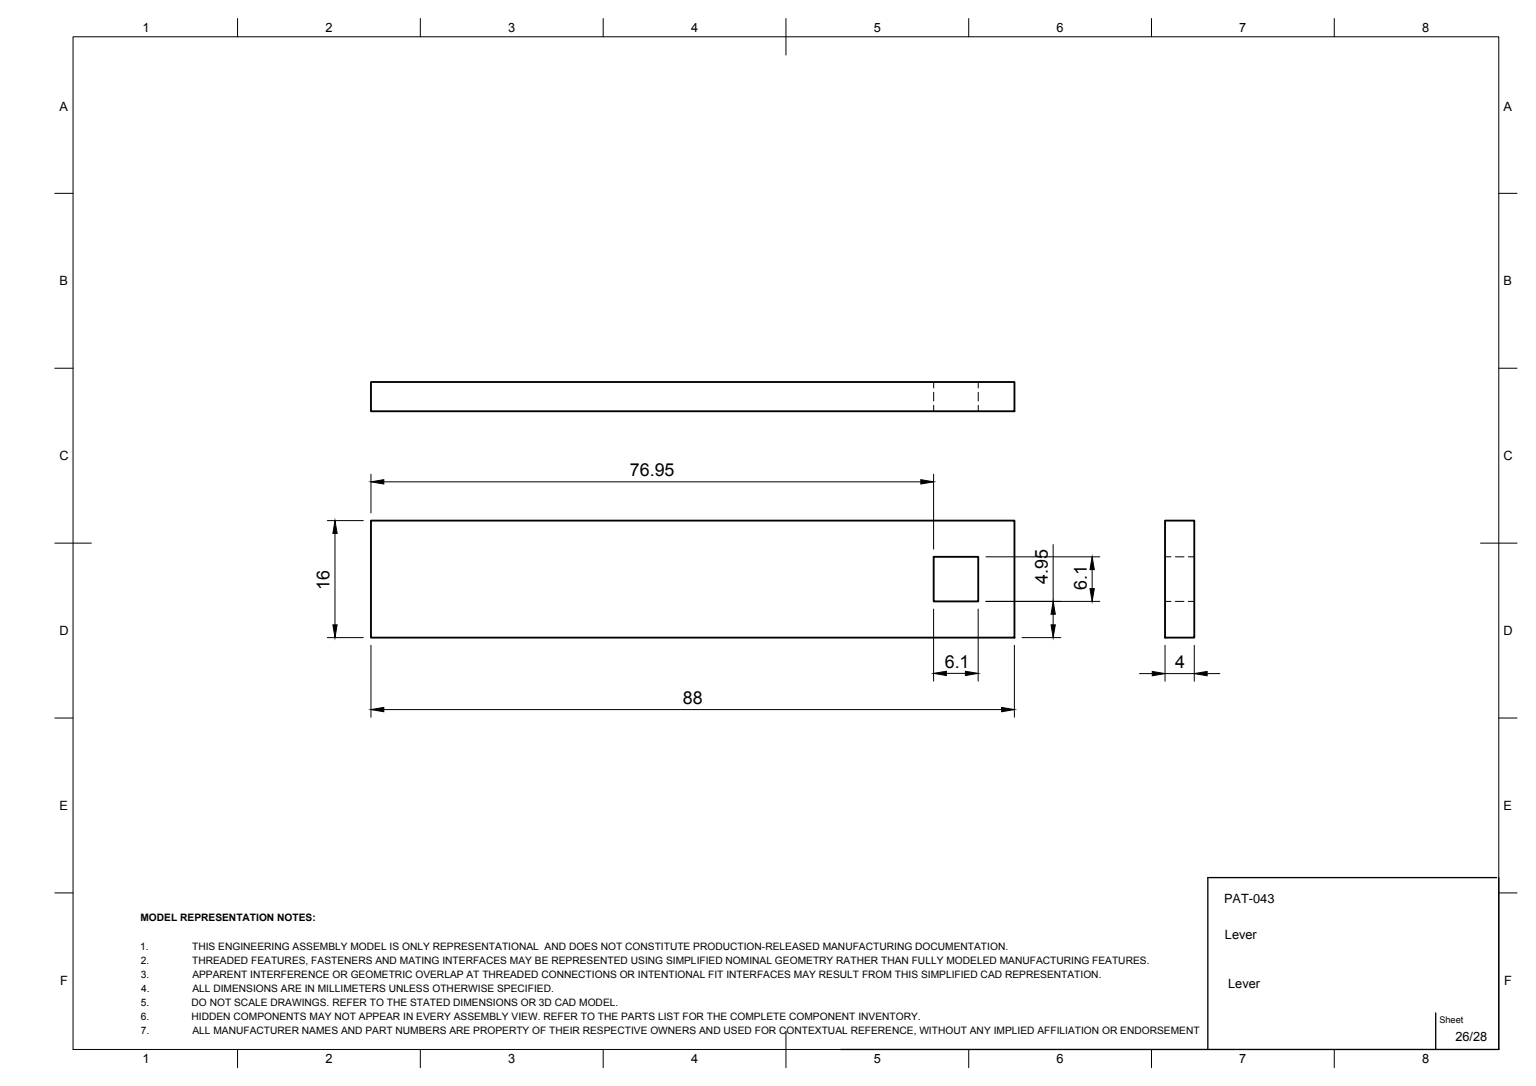
ISO-10303-21;
HEADER;
/* Generated by software containing ST-Developer
 * from STEP Tools, Inc. (www.steptools.com) 
 */

FILE_DESCRIPTION(
/* description */ ('Four-valve pipe header'),
/* implementation_level */ '2;1');

FILE_NAME(
/* name */ 'Lever.step',
/* time_stamp */ '2026-10-29T16:56:19-07:00',
/* author */ (''),
/* organization */ (''),
/* preprocessor_version */ 'ST-DEVELOPER v20.2',
/* originating_system */ 'Autodesk Translation Framework v15.17.0.0',
/* authorisation */ '');

FILE_SCHEMA (('AUTOMOTIVE_DESIGN { 1 0 10303 214 3 1 1 }'));
ENDSEC;

DATA;
#10=MECHANICAL_DESIGN_GEOMETRIC_PRESENTATION_REPRESENTATION('',(#355),#10119);
#303=SHAPE_REPRESENTATION_RELATIONSHIP('SRR','None',#10266,#329);
#329=ADVANCED_BREP_SHAPE_REPRESENTATION('',(#379),#10115);
#355=STYLED_ITEM('',(#10484),#379);
#379=MANIFOLD_SOLID_BREP('Body1',#5603);
#530=FACE_BOUND('',#1488,.T.);
#531=FACE_BOUND('',#1490,.T.);
#718=PLANE('',#6463);
#719=PLANE('',#6464);
#720=PLANE('',#6465);
#721=PLANE('',#6466);
#722=PLANE('',#6467);
#723=PLANE('',#6468);
#724=PLANE('',#6469);
#725=PLANE('',#6470);
#726=PLANE('',#6471);
#727=PLANE('',#6472);
#1043=FACE_OUTER_BOUND('',#1479,.T.);
#1044=FACE_OUTER_BOUND('',#1480,.T.);
#1045=FACE_OUTER_BOUND('',#1481,.T.);
#1046=FACE_OUTER_BOUND('',#1482,.T.);
#1047=FACE_OUTER_BOUND('',#1483,.T.);
#1048=FACE_OUTER_BOUND('',#1484,.T.);
#1049=FACE_OUTER_BOUND('',#1485,.T.);
#1050=FACE_OUTER_BOUND('',#1486,.T.);
#1051=FACE_OUTER_BOUND('',#1487,.T.);
#1052=FACE_OUTER_BOUND('',#1489,.T.);
#1479=EDGE_LOOP('',(#5005,#5006,#5007,#5008));
#1480=EDGE_LOOP('',(#5009,#5010,#5011,#5012));
#1481=EDGE_LOOP('',(#5013,#5014,#5015,#5016));
#1482=EDGE_LOOP('',(#5017,#5018,#5019,#5020));
#1483=EDGE_LOOP('',(#5021,#5022,#5023,#5024));
#1484=EDGE_LOOP('',(#5025,#5026,#5027,#5028));
#1485=EDGE_LOOP('',(#5029,#5030,#5031,#5032));
#1486=EDGE_LOOP('',(#5033,#5034,#5035,#5036));
#1487=EDGE_LOOP('',(#5037,#5038,#5039,#5040));
#1488=EDGE_LOOP('',(#5041,#5042,#5043,#5044));
#1489=EDGE_LOOP('',(#5045,#5046,#5047,#5048));
#1490=EDGE_LOOP('',(#5049,#5050,#5051,#5052));
#1877=LINE('',#9847,#2295);
#1878=LINE('',#9849,#2296);
#1879=LINE('',#9851,#2297);
#1880=LINE('',#9852,#2298);
#1881=LINE('',#9855,#2299);
#1882=LINE('',#9857,#2300);
#1883=LINE('',#9858,#2301);
#1884=LINE('',#9861,#2302);
#1885=LINE('',#9863,#2303);
#1886=LINE('',#9864,#2304);
#1887=LINE('',#9866,#2305);
#1888=LINE('',#9867,#2306);
#1889=LINE('',#9871,#2307);
#1890=LINE('',#9873,#2308);
#1891=LINE('',#9875,#2309);
#1892=LINE('',#9876,#2310);
#1893=LINE('',#9879,#2311);
#1894=LINE('',#9881,#2312);
#1895=LINE('',#9882,#2313);
#1896=LINE('',#9885,#2314);
#1897=LINE('',#9887,#2315);
#1898=LINE('',#9888,#2316);
#1899=LINE('',#9890,#2317);
#1900=LINE('',#9891,#2318);
#2295=VECTOR('',#8064,1.);
#2296=VECTOR('',#8065,1.);
#2297=VECTOR('',#8066,1.);
#2298=VECTOR('',#8067,1.);
#2299=VECTOR('',#8070,1.);
#2300=VECTOR('',#8071,1.);
#2301=VECTOR('',#8072,1.);
#2302=VECTOR('',#8075,1.);
#2303=VECTOR('',#8076,1.);
#2304=VECTOR('',#8077,1.);
#2305=VECTOR('',#8080,1.);
#2306=VECTOR('',#8081,1.);
#2307=VECTOR('',#8084,1.);
#2308=VECTOR('',#8085,1.);
#2309=VECTOR('',#8086,1.);
#2310=VECTOR('',#8087,1.);
#2311=VECTOR('',#8090,1.);
#2312=VECTOR('',#8091,1.);
#2313=VECTOR('',#8092,1.);
#2314=VECTOR('',#8095,1.);
#2315=VECTOR('',#8096,1.);
#2316=VECTOR('',#8097,1.);
#2317=VECTOR('',#8100,1.);
#2318=VECTOR('',#8101,1.);
#2990=VERTEX_POINT('',#9845);
#2991=VERTEX_POINT('',#9846);
#2992=VERTEX_POINT('',#9848);
#2993=VERTEX_POINT('',#9850);
#2994=VERTEX_POINT('',#9854);
#2995=VERTEX_POINT('',#9856);
#2996=VERTEX_POINT('',#9860);
#2997=VERTEX_POINT('',#9862);
#2998=VERTEX_POINT('',#9869);
#2999=VERTEX_POINT('',#9870);
#3000=VERTEX_POINT('',#9872);
#3001=VERTEX_POINT('',#9874);
#3002=VERTEX_POINT('',#9878);
#3003=VERTEX_POINT('',#9880);
#3004=VERTEX_POINT('',#9884);
#3005=VERTEX_POINT('',#9886);
#3669=EDGE_CURVE('',#2990,#2991,#1877,.T.);
#3670=EDGE_CURVE('',#2992,#2990,#1878,.T.);
#3671=EDGE_CURVE('',#2993,#2992,#1879,.T.);
#3672=EDGE_CURVE('',#2993,#2991,#1880,.T.);
#3673=EDGE_CURVE('',#2991,#2994,#1881,.T.);
#3674=EDGE_CURVE('',#2995,#2993,#1882,.T.);
#3675=EDGE_CURVE('',#2995,#2994,#1883,.T.);
#3676=EDGE_CURVE('',#2994,#2996,#1884,.T.);
#3677=EDGE_CURVE('',#2997,#2995,#1885,.T.);
#3678=EDGE_CURVE('',#2997,#2996,#1886,.T.);
#3679=EDGE_CURVE('',#2996,#2990,#1887,.T.);
#3680=EDGE_CURVE('',#2992,#2997,#1888,.T.);
#3681=EDGE_CURVE('',#2998,#2999,#1889,.T.);
#3682=EDGE_CURVE('',#2999,#3000,#1890,.T.);
#3683=EDGE_CURVE('',#3001,#3000,#1891,.T.);
#3684=EDGE_CURVE('',#2998,#3001,#1892,.T.);
#3685=EDGE_CURVE('',#3002,#2998,#1893,.T.);
#3686=EDGE_CURVE('',#3003,#3001,#1894,.T.);
#3687=EDGE_CURVE('',#3002,#3003,#1895,.T.);
#3688=EDGE_CURVE('',#3004,#3002,#1896,.T.);
#3689=EDGE_CURVE('',#3005,#3003,#1897,.T.);
#3690=EDGE_CURVE('',#3004,#3005,#1898,.T.);
#3691=EDGE_CURVE('',#2999,#3004,#1899,.T.);
#3692=EDGE_CURVE('',#3000,#3005,#1900,.T.);
#5005=ORIENTED_EDGE('',*,*,#3669,.F.);
#5006=ORIENTED_EDGE('',*,*,#3670,.F.);
#5007=ORIENTED_EDGE('',*,*,#3671,.F.);
#5008=ORIENTED_EDGE('',*,*,#3672,.T.);
#5009=ORIENTED_EDGE('',*,*,#3673,.F.);
#5010=ORIENTED_EDGE('',*,*,#3672,.F.);
#5011=ORIENTED_EDGE('',*,*,#3674,.F.);
#5012=ORIENTED_EDGE('',*,*,#3675,.T.);
#5013=ORIENTED_EDGE('',*,*,#3676,.F.);
#5014=ORIENTED_EDGE('',*,*,#3675,.F.);
#5015=ORIENTED_EDGE('',*,*,#3677,.F.);
#5016=ORIENTED_EDGE('',*,*,#3678,.T.);
#5017=ORIENTED_EDGE('',*,*,#3679,.F.);
#5018=ORIENTED_EDGE('',*,*,#3678,.F.);
#5019=ORIENTED_EDGE('',*,*,#3680,.F.);
#5020=ORIENTED_EDGE('',*,*,#3670,.T.);
#5021=ORIENTED_EDGE('',*,*,#3681,.T.);
#5022=ORIENTED_EDGE('',*,*,#3682,.T.);
#5023=ORIENTED_EDGE('',*,*,#3683,.F.);
#5024=ORIENTED_EDGE('',*,*,#3684,.F.);
#5025=ORIENTED_EDGE('',*,*,#3685,.T.);
#5026=ORIENTED_EDGE('',*,*,#3684,.T.);
#5027=ORIENTED_EDGE('',*,*,#3686,.F.);
#5028=ORIENTED_EDGE('',*,*,#3687,.F.);
#5029=ORIENTED_EDGE('',*,*,#3688,.T.);
#5030=ORIENTED_EDGE('',*,*,#3687,.T.);
#5031=ORIENTED_EDGE('',*,*,#3689,.F.);
#5032=ORIENTED_EDGE('',*,*,#3690,.F.);
#5033=ORIENTED_EDGE('',*,*,#3691,.T.);
#5034=ORIENTED_EDGE('',*,*,#3690,.T.);
#5035=ORIENTED_EDGE('',*,*,#3692,.F.);
#5036=ORIENTED_EDGE('',*,*,#3682,.F.);
#5037=ORIENTED_EDGE('',*,*,#3692,.T.);
#5038=ORIENTED_EDGE('',*,*,#3689,.T.);
#5039=ORIENTED_EDGE('',*,*,#3686,.T.);
#5040=ORIENTED_EDGE('',*,*,#3683,.T.);
#5041=ORIENTED_EDGE('',*,*,#3676,.T.);
#5042=ORIENTED_EDGE('',*,*,#3679,.T.);
#5043=ORIENTED_EDGE('',*,*,#3669,.T.);
#5044=ORIENTED_EDGE('',*,*,#3673,.T.);
#5045=ORIENTED_EDGE('',*,*,#3691,.F.);
#5046=ORIENTED_EDGE('',*,*,#3681,.F.);
#5047=ORIENTED_EDGE('',*,*,#3685,.F.);
#5048=ORIENTED_EDGE('',*,*,#3688,.F.);
#5049=ORIENTED_EDGE('',*,*,#3677,.T.);
#5050=ORIENTED_EDGE('',*,*,#3674,.T.);
#5051=ORIENTED_EDGE('',*,*,#3671,.T.);
#5052=ORIENTED_EDGE('',*,*,#3680,.T.);
#5543=ADVANCED_FACE('',(#1043),#718,.F.);
#5544=ADVANCED_FACE('',(#1044),#719,.F.);
#5545=ADVANCED_FACE('',(#1045),#720,.F.);
#5546=ADVANCED_FACE('',(#1046),#721,.F.);
#5547=ADVANCED_FACE('',(#1047),#722,.T.);
#5548=ADVANCED_FACE('',(#1048),#723,.T.);
#5549=ADVANCED_FACE('',(#1049),#724,.T.);
#5550=ADVANCED_FACE('',(#1050),#725,.T.);
#5551=ADVANCED_FACE('',(#1051,#530),#726,.T.);
#5552=ADVANCED_FACE('',(#1052,#531),#727,.F.);
#5603=CLOSED_SHELL('',(#5543,#5544,#5545,#5546,#5547,#5548,#5549,#5550,
#5551,#5552));
#6462=AXIS2_PLACEMENT_3D('',#9843,#8060,#8061);
#6463=AXIS2_PLACEMENT_3D('',#9844,#8062,#8063);
#6464=AXIS2_PLACEMENT_3D('',#9853,#8068,#8069);
#6465=AXIS2_PLACEMENT_3D('',#9859,#8073,#8074);
#6466=AXIS2_PLACEMENT_3D('',#9865,#8078,#8079);
#6467=AXIS2_PLACEMENT_3D('',#9868,#8082,#8083);
#6468=AXIS2_PLACEMENT_3D('',#9877,#8088,#8089);
#6469=AXIS2_PLACEMENT_3D('',#9883,#8093,#8094);
#6470=AXIS2_PLACEMENT_3D('',#9889,#8098,#8099);
#6471=AXIS2_PLACEMENT_3D('',#9892,#8102,#8103);
#6472=AXIS2_PLACEMENT_3D('',#9893,#8104,#8105);
#8060=DIRECTION('axis',(0.,0.,1.));
#8061=DIRECTION('refdir',(1.,0.,0.));
#8062=DIRECTION('center_axis',(0.,-1.,0.));
#8063=DIRECTION('ref_axis',(1.,0.,0.));
#8064=DIRECTION('',(-1.,0.,0.));
#8065=DIRECTION('',(0.,0.,1.));
#8066=DIRECTION('',(1.,0.,0.));
#8067=DIRECTION('',(0.,0.,1.));
#8068=DIRECTION('center_axis',(-1.,0.,0.));
#8069=DIRECTION('ref_axis',(0.,-1.,0.));
#8070=DIRECTION('',(0.,1.,0.));
#8071=DIRECTION('',(0.,-1.,0.));
#8072=DIRECTION('',(0.,0.,1.));
#8073=DIRECTION('center_axis',(0.,1.,0.));
#8074=DIRECTION('ref_axis',(-1.,0.,0.));
#8075=DIRECTION('',(1.,0.,0.));
#8076=DIRECTION('',(-1.,0.,0.));
#8077=DIRECTION('',(0.,0.,1.));
#8078=DIRECTION('center_axis',(1.,0.,0.));
#8079=DIRECTION('ref_axis',(0.,1.,0.));
#8080=DIRECTION('',(0.,-1.,0.));
#8081=DIRECTION('',(0.,1.,0.));
#8082=DIRECTION('center_axis',(0.,1.,0.));
#8083=DIRECTION('ref_axis',(-1.,0.,0.));
#8084=DIRECTION('',(-1.,0.,0.));
#8085=DIRECTION('',(0.,0.,1.));
#8086=DIRECTION('',(-1.,0.,0.));
#8087=DIRECTION('',(0.,0.,1.));
#8088=DIRECTION('center_axis',(1.,0.,0.));
#8089=DIRECTION('ref_axis',(0.,1.,0.));
#8090=DIRECTION('',(0.,1.,0.));
#8091=DIRECTION('',(0.,1.,0.));
#8092=DIRECTION('',(0.,0.,1.));
#8093=DIRECTION('center_axis',(0.,-1.,0.));
#8094=DIRECTION('ref_axis',(1.,0.,0.));
#8095=DIRECTION('',(1.,0.,0.));
#8096=DIRECTION('',(1.,0.,0.));
#8097=DIRECTION('',(0.,0.,1.));
#8098=DIRECTION('center_axis',(-1.,0.,0.));
#8099=DIRECTION('ref_axis',(0.,-1.,0.));
#8100=DIRECTION('',(0.,-1.,0.));
#8101=DIRECTION('',(0.,-1.,0.));
#8102=DIRECTION('center_axis',(0.,0.,1.));
#8103=DIRECTION('ref_axis',(1.,0.,0.));
#8104=DIRECTION('center_axis',(0.,0.,1.));
#8105=DIRECTION('ref_axis',(1.,0.,0.));
#9843=CARTESIAN_POINT('',(0.,0.,0.));
#9844=CARTESIAN_POINT('Origin',(-0.305,-0.305,8.9));
#9845=CARTESIAN_POINT('',(0.305,-0.305,9.4));
#9846=CARTESIAN_POINT('',(-0.305,-0.305,9.4));
#9847=CARTESIAN_POINT('',(1.6475,-0.305,9.4));
#9848=CARTESIAN_POINT('',(0.305,-0.305,9.));
#9849=CARTESIAN_POINT('',(0.305,-0.305,8.9));
#9850=CARTESIAN_POINT('',(-0.305,-0.305,9.));
#9851=CARTESIAN_POINT('',(1.6475,-0.305,9.));
#9852=CARTESIAN_POINT('',(-0.305,-0.305,8.9));
#9853=CARTESIAN_POINT('Origin',(-0.305,0.305,8.9));
#9854=CARTESIAN_POINT('',(-0.305,0.305,9.4));
#9855=CARTESIAN_POINT('',(-0.305,0.1525,9.4));
#9856=CARTESIAN_POINT('',(-0.305,0.305,9.));
#9857=CARTESIAN_POINT('',(-0.305,0.1525,9.));
#9858=CARTESIAN_POINT('',(-0.305,0.305,8.9));
#9859=CARTESIAN_POINT('Origin',(0.305,0.305,8.9));
#9860=CARTESIAN_POINT('',(0.305,0.305,9.4));
#9861=CARTESIAN_POINT('',(1.9525,0.305,9.4));
#9862=CARTESIAN_POINT('',(0.305,0.305,9.));
#9863=CARTESIAN_POINT('',(1.9525,0.305,9.));
#9864=CARTESIAN_POINT('',(0.305,0.305,8.9));
#9865=CARTESIAN_POINT('Origin',(0.305,-0.305,8.9));
#9866=CARTESIAN_POINT('',(0.305,-0.1525,9.4));
#9867=CARTESIAN_POINT('',(0.305,-0.1525,9.));
#9868=CARTESIAN_POINT('Origin',(8.,0.8,9.));
#9869=CARTESIAN_POINT('',(8.,0.8,9.));
#9870=CARTESIAN_POINT('',(-0.8,0.8,9.));
#9871=CARTESIAN_POINT('',(8.,0.8,9.));
#9872=CARTESIAN_POINT('',(-0.8,0.8,9.4));
#9873=CARTESIAN_POINT('',(-0.8,0.8,9.));
#9874=CARTESIAN_POINT('',(8.,0.8,9.4));
#9875=CARTESIAN_POINT('',(8.,0.8,9.4));
#9876=CARTESIAN_POINT('',(8.,0.8,9.));
#9877=CARTESIAN_POINT('Origin',(8.,-0.8,9.));
#9878=CARTESIAN_POINT('',(8.,-0.8,9.));
#9879=CARTESIAN_POINT('',(8.,-0.8,9.));
#9880=CARTESIAN_POINT('',(8.,-0.8,9.4));
#9881=CARTESIAN_POINT('',(8.,-0.8,9.4));
#9882=CARTESIAN_POINT('',(8.,-0.8,9.));
#9883=CARTESIAN_POINT('Origin',(-0.8,-0.8,9.));
#9884=CARTESIAN_POINT('',(-0.8,-0.8,9.));
#9885=CARTESIAN_POINT('',(-0.8,-0.8,9.));
#9886=CARTESIAN_POINT('',(-0.8,-0.8,9.4));
#9887=CARTESIAN_POINT('',(-0.8,-0.8,9.4));
#9888=CARTESIAN_POINT('',(-0.8,-0.8,9.));
#9889=CARTESIAN_POINT('Origin',(-0.8,0.8,9.));
#9890=CARTESIAN_POINT('',(-0.8,0.8,9.));
#9891=CARTESIAN_POINT('',(-0.8,0.8,9.4));
#9892=CARTESIAN_POINT('Origin',(3.6,0.,9.4));
#9893=CARTESIAN_POINT('Origin',(3.6,0.,9.));
#10084=UNCERTAINTY_MEASURE_WITH_UNIT(LENGTH_MEASURE(0.001),#10120,
'DISTANCE_ACCURACY_VALUE',
'Maximum model space distance between geometric entities at asserted c
onnectivities');
#10088=UNCERTAINTY_MEASURE_WITH_UNIT(LENGTH_MEASURE(0.001),#10120,
'DISTANCE_ACCURACY_VALUE',
'Maximum model space distance between geometric entities at asserted c
onnectivities');
#10115=(
GEOMETRIC_REPRESENTATION_CONTEXT(3)
GLOBAL_UNCERTAINTY_ASSIGNED_CONTEXT((#10084))
GLOBAL_UNIT_ASSIGNED_CONTEXT((#10120,#10122,#10123))
REPRESENTATION_CONTEXT('','3D')
);
#10119=(
GEOMETRIC_REPRESENTATION_CONTEXT(3)
GLOBAL_UNCERTAINTY_ASSIGNED_CONTEXT((#10088))
GLOBAL_UNIT_ASSIGNED_CONTEXT((#10120,#10122,#10123))
REPRESENTATION_CONTEXT('','3D')
);
#10120=(
LENGTH_UNIT()
NAMED_UNIT(*)
SI_UNIT(.CENTI.,.METRE.)
);
#10122=(
NAMED_UNIT(*)
PLANE_ANGLE_UNIT()
SI_UNIT($,.RADIAN.)
);
#10123=(
NAMED_UNIT(*)
SI_UNIT($,.STERADIAN.)
SOLID_ANGLE_UNIT()
);
#10150=SHAPE_DEFINITION_REPRESENTATION(#10180,#10266);
#10180=PRODUCT_DEFINITION_SHAPE('',$,#10297);
#10266=SHAPE_REPRESENTATION('',(#6462),#10115);
#10270=PRODUCT_DEFINITION_CONTEXT('part definition',#10362,'design');
#10297=PRODUCT_DEFINITION('Lever','Lever',#10327,#10270);
#10327=PRODUCT_DEFINITION_FORMATION('',$,#10390);
#10362=APPLICATION_CONTEXT(
'Core Data for Automotive Mechanical Design Process');
#10363=PRODUCT_CONTEXT('part definition',#10362,'mechanical');
#10390=PRODUCT('Lever','Lever',
'Lever',(#10363));
#10478=COLOUR_RGB('Off White',0.89,0.88,0.83);
#10479=FILL_AREA_STYLE_COLOUR('',#10478);
#10480=FILL_AREA_STYLE('',(#10479));
#10481=SURFACE_STYLE_FILL_AREA(#10480);
#10482=SURFACE_SIDE_STYLE('',(#10481));
#10483=SURFACE_STYLE_USAGE(.BOTH.,#10482);
#10484=PRESENTATION_STYLE_ASSIGNMENT((#10483));
ENDSEC;
END-ISO-10303-21;
